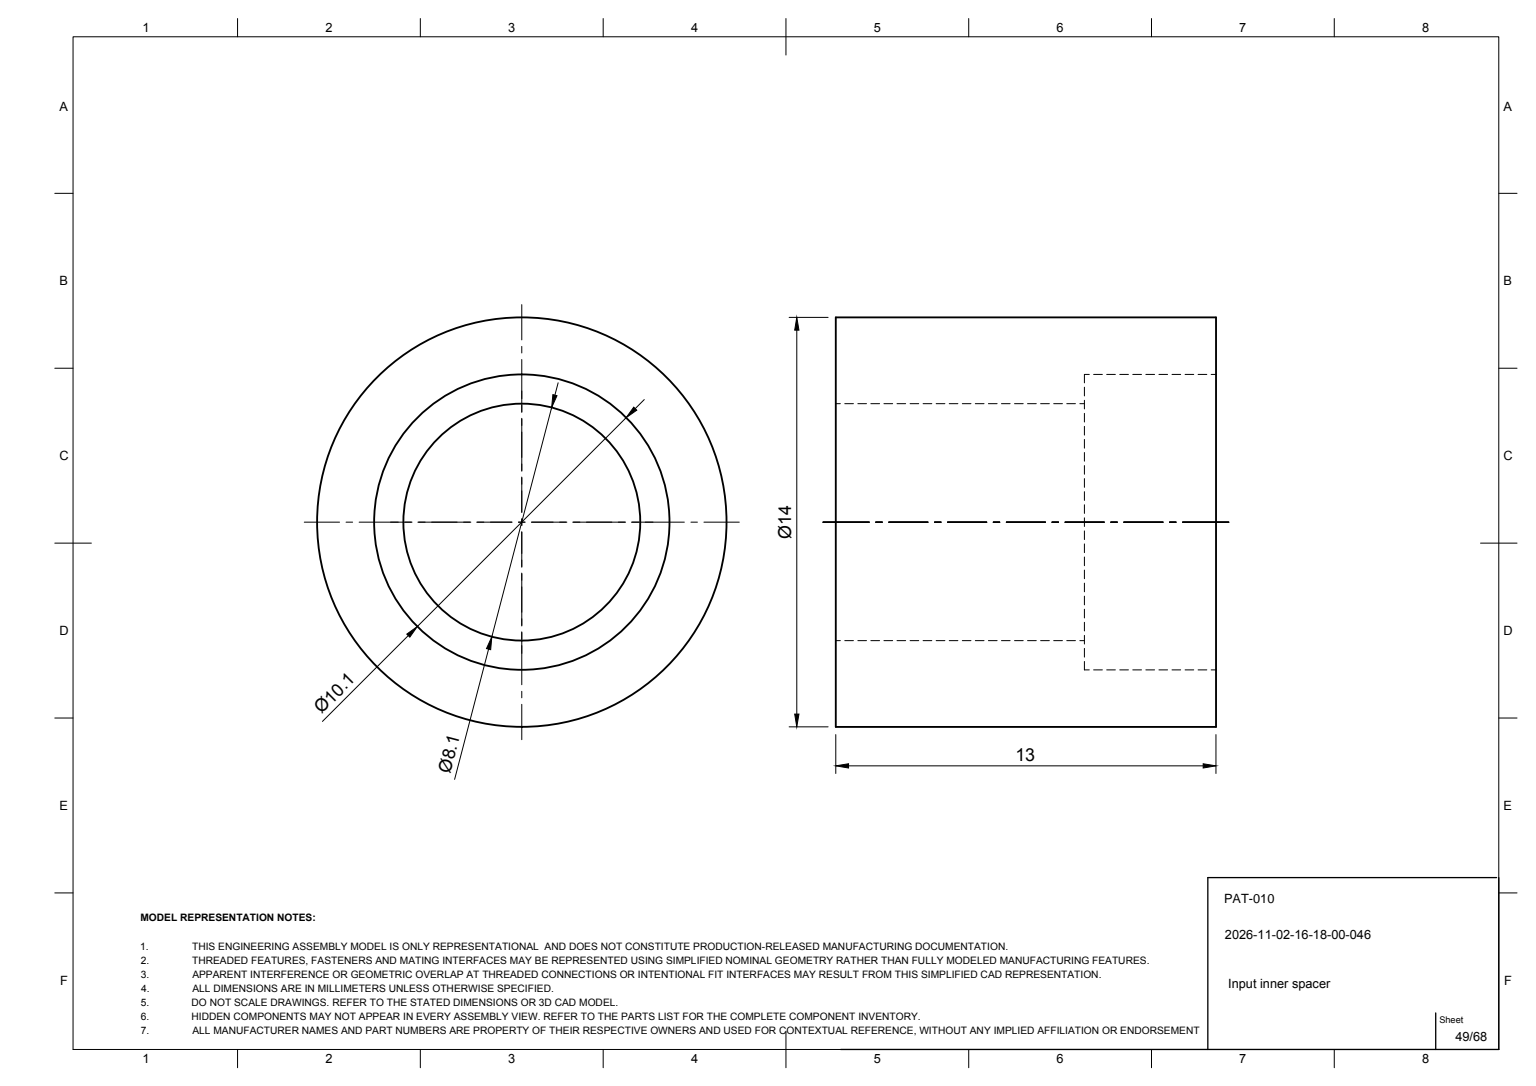
ISO-10303-21;
HEADER;
/* Generated by software containing ST-Developer
 * from STEP Tools, Inc. (www.steptools.com) 
 */

FILE_DESCRIPTION(
/* description */ ('Belt conveyor head drive unit'),
/* implementation_level */ '2;1');

FILE_NAME(
/* name */ 'Input inner spacer.step',
/* time_stamp */ '2026-10-28T03:26:19-07:00',
/* author */ (''),
/* organization */ (''),
/* preprocessor_version */ 'ST-DEVELOPER v20.2',
/* originating_system */ 'Autodesk Translation Framework v15.17.0.0',
/* authorisation */ '');

FILE_SCHEMA (('AUTOMOTIVE_DESIGN { 1 0 10303 214 3 1 1 }'));
ENDSEC;

DATA;
#10=MECHANICAL_DESIGN_GEOMETRIC_PRESENTATION_REPRESENTATION('',(#908),#27069);
#754=SHAPE_REPRESENTATION_RELATIONSHIP('SRR','None',#27402,#823);
#823=ADVANCED_BREP_SHAPE_REPRESENTATION('',(#989),#27044);
#908=STYLED_ITEM('',(#27811),#989);
#989=MANIFOLD_SOLID_BREP('Body1',#13777);
#1209=FACE_BOUND('',#3157,.T.);
#1210=FACE_BOUND('',#3161,.T.);
#1211=FACE_BOUND('',#3163,.T.);
#1547=PLANE('',#15663);
#1548=PLANE('',#15670);
#1549=PLANE('',#15671);
#2158=FACE_OUTER_BOUND('',#3155,.T.);
#2159=FACE_OUTER_BOUND('',#3156,.T.);
#2160=FACE_OUTER_BOUND('',#3158,.T.);
#2161=FACE_OUTER_BOUND('',#3159,.T.);
#2162=FACE_OUTER_BOUND('',#3160,.T.);
#2163=FACE_OUTER_BOUND('',#3162,.T.);
#3155=EDGE_LOOP('',(#11190,#11191,#11192,#11193));
#3156=EDGE_LOOP('',(#11194));
#3157=EDGE_LOOP('',(#11195));
#3158=EDGE_LOOP('',(#11196,#11197,#11198,#11199));
#3159=EDGE_LOOP('',(#11200,#11201,#11202,#11203));
#3160=EDGE_LOOP('',(#11204));
#3161=EDGE_LOOP('',(#11205));
#3162=EDGE_LOOP('',(#11206));
#3163=EDGE_LOOP('',(#11207));
#4049=LINE('',#24483,#4841);
#4050=LINE('',#24490,#4842);
#4051=LINE('',#24496,#4843);
#4841=VECTOR('',#19185,0.505);
#4842=VECTOR('',#19194,0.405);
#4843=VECTOR('',#19201,0.7);
#5591=CIRCLE('',#15661,0.505);
#5592=CIRCLE('',#15662,0.505);
#5593=CIRCLE('',#15664,0.405);
#5594=CIRCLE('',#15666,0.405);
#5595=CIRCLE('',#15668,0.7);
#5596=CIRCLE('',#15669,0.7);
#6717=VERTEX_POINT('',#24480);
#6718=VERTEX_POINT('',#24482);
#6719=VERTEX_POINT('',#24486);
#6720=VERTEX_POINT('',#24489);
#6721=VERTEX_POINT('',#24493);
#6722=VERTEX_POINT('',#24495);
#8287=EDGE_CURVE('',#6717,#6717,#5591,.T.);
#8288=EDGE_CURVE('',#6717,#6718,#4049,.T.);
#8289=EDGE_CURVE('',#6718,#6718,#5592,.T.);
#8290=EDGE_CURVE('',#6719,#6719,#5593,.T.);
#8291=EDGE_CURVE('',#6719,#6720,#4050,.T.);
#8292=EDGE_CURVE('',#6720,#6720,#5594,.T.);
#8293=EDGE_CURVE('',#6721,#6721,#5595,.T.);
#8294=EDGE_CURVE('',#6721,#6722,#4051,.T.);
#8295=EDGE_CURVE('',#6722,#6722,#5596,.T.);
#11190=ORIENTED_EDGE('',*,*,#8287,.F.);
#11191=ORIENTED_EDGE('',*,*,#8288,.T.);
#11192=ORIENTED_EDGE('',*,*,#8289,.F.);
#11193=ORIENTED_EDGE('',*,*,#8288,.F.);
#11194=ORIENTED_EDGE('',*,*,#8287,.T.);
#11195=ORIENTED_EDGE('',*,*,#8290,.F.);
#11196=ORIENTED_EDGE('',*,*,#8290,.T.);
#11197=ORIENTED_EDGE('',*,*,#8291,.T.);
#11198=ORIENTED_EDGE('',*,*,#8292,.T.);
#11199=ORIENTED_EDGE('',*,*,#8291,.F.);
#11200=ORIENTED_EDGE('',*,*,#8293,.F.);
#11201=ORIENTED_EDGE('',*,*,#8294,.T.);
#11202=ORIENTED_EDGE('',*,*,#8295,.T.);
#11203=ORIENTED_EDGE('',*,*,#8294,.F.);
#11204=ORIENTED_EDGE('',*,*,#8293,.T.);
#11205=ORIENTED_EDGE('',*,*,#8289,.T.);
#11206=ORIENTED_EDGE('',*,*,#8295,.F.);
#11207=ORIENTED_EDGE('',*,*,#8292,.F.);
#12729=CYLINDRICAL_SURFACE('',#15660,0.505);
#12730=CYLINDRICAL_SURFACE('',#15665,0.405);
#12731=CYLINDRICAL_SURFACE('',#15667,0.7);
#13437=ADVANCED_FACE('',(#2158),#12729,.F.);
#13438=ADVANCED_FACE('',(#2159,#1209),#1547,.T.);
#13439=ADVANCED_FACE('',(#2160),#12730,.F.);
#13440=ADVANCED_FACE('',(#2161),#12731,.T.);
#13441=ADVANCED_FACE('',(#2162,#1210),#1548,.T.);
#13442=ADVANCED_FACE('',(#2163,#1211),#1549,.F.);
#13777=CLOSED_SHELL('',(#13437,#13438,#13439,#13440,#13441,#13442));
#15659=AXIS2_PLACEMENT_3D('',#24478,#19179,#19180);
#15660=AXIS2_PLACEMENT_3D('',#24479,#19181,#19182);
#15661=AXIS2_PLACEMENT_3D('',#24481,#19183,#19184);
#15662=AXIS2_PLACEMENT_3D('',#24484,#19186,#19187);
#15663=AXIS2_PLACEMENT_3D('',#24485,#19188,#19189);
#15664=AXIS2_PLACEMENT_3D('',#24487,#19190,#19191);
#15665=AXIS2_PLACEMENT_3D('',#24488,#19192,#19193);
#15666=AXIS2_PLACEMENT_3D('',#24491,#19195,#19196);
#15667=AXIS2_PLACEMENT_3D('',#24492,#19197,#19198);
#15668=AXIS2_PLACEMENT_3D('',#24494,#19199,#19200);
#15669=AXIS2_PLACEMENT_3D('',#24497,#19202,#19203);
#15670=AXIS2_PLACEMENT_3D('',#24498,#19204,#19205);
#15671=AXIS2_PLACEMENT_3D('',#24499,#19206,#19207);
#19179=DIRECTION('axis',(0.,0.,1.));
#19180=DIRECTION('refdir',(1.,0.,0.));
#19181=DIRECTION('center_axis',(0.,1.,0.));
#19182=DIRECTION('ref_axis',(1.,0.,0.));
#19183=DIRECTION('center_axis',(0.,1.,0.));
#19184=DIRECTION('ref_axis',(1.,0.,0.));
#19185=DIRECTION('',(0.,1.,0.));
#19186=DIRECTION('center_axis',(0.,-1.,0.));
#19187=DIRECTION('ref_axis',(1.,0.,0.));
#19188=DIRECTION('center_axis',(0.,1.,0.));
#19189=DIRECTION('ref_axis',(1.,0.,0.));
#19190=DIRECTION('center_axis',(0.,1.,0.));
#19191=DIRECTION('ref_axis',(1.,0.,0.));
#19192=DIRECTION('center_axis',(0.,1.,0.));
#19193=DIRECTION('ref_axis',(1.,0.,0.));
#19194=DIRECTION('',(0.,-1.,0.));
#19195=DIRECTION('center_axis',(0.,-1.,0.));
#19196=DIRECTION('ref_axis',(1.,0.,0.));
#19197=DIRECTION('center_axis',(0.,1.,0.));
#19198=DIRECTION('ref_axis',(1.,0.,0.));
#19199=DIRECTION('center_axis',(0.,1.,0.));
#19200=DIRECTION('ref_axis',(1.,0.,0.));
#19201=DIRECTION('',(0.,-1.,0.));
#19202=DIRECTION('center_axis',(0.,1.,0.));
#19203=DIRECTION('ref_axis',(1.,0.,0.));
#19204=DIRECTION('center_axis',(0.,1.,0.));
#19205=DIRECTION('ref_axis',(1.,0.,0.));
#19206=DIRECTION('center_axis',(0.,1.,0.));
#19207=DIRECTION('ref_axis',(1.,0.,0.));
#24478=CARTESIAN_POINT('',(0.,0.,0.));
#24479=CARTESIAN_POINT('Origin',(0.,-1.8,7.));
#24480=CARTESIAN_POINT('',(-0.505,-1.8,7.));
#24481=CARTESIAN_POINT('Origin',(0.,-1.8,7.));
#24482=CARTESIAN_POINT('',(-0.505,-1.35,7.));
#24483=CARTESIAN_POINT('',(-0.505,-1.8,7.));
#24484=CARTESIAN_POINT('Origin',(0.,-1.35,7.));
#24485=CARTESIAN_POINT('Origin',(0.,-1.8,7.));
#24486=CARTESIAN_POINT('',(-0.405,-1.8,7.));
#24487=CARTESIAN_POINT('Origin',(0.,-1.8,7.));
#24488=CARTESIAN_POINT('Origin',(0.,-2.65,7.));
#24489=CARTESIAN_POINT('',(-0.405,-2.65,7.));
#24490=CARTESIAN_POINT('',(-0.405,-2.65,7.));
#24491=CARTESIAN_POINT('Origin',(0.,-2.65,7.));
#24492=CARTESIAN_POINT('Origin',(0.,-2.65,7.));
#24493=CARTESIAN_POINT('',(-0.7,-1.35,7.));
#24494=CARTESIAN_POINT('Origin',(0.,-1.35,7.));
#24495=CARTESIAN_POINT('',(-0.7,-2.65,7.));
#24496=CARTESIAN_POINT('',(-0.7,-2.65,7.));
#24497=CARTESIAN_POINT('Origin',(0.,-2.65,7.));
#24498=CARTESIAN_POINT('Origin',(0.,-1.35,7.));
#24499=CARTESIAN_POINT('Origin',(0.,-2.65,7.));
#26967=UNCERTAINTY_MEASURE_WITH_UNIT(LENGTH_MEASURE(0.001),#27070,
'DISTANCE_ACCURACY_VALUE',
'Maximum model space distance between geometric entities at asserted c
onnectivities');
#26992=UNCERTAINTY_MEASURE_WITH_UNIT(LENGTH_MEASURE(0.001),#27070,
'DISTANCE_ACCURACY_VALUE',
'Maximum model space distance between geometric entities at asserted c
onnectivities');
#27044=(
GEOMETRIC_REPRESENTATION_CONTEXT(3)
GLOBAL_UNCERTAINTY_ASSIGNED_CONTEXT((#26967))
GLOBAL_UNIT_ASSIGNED_CONTEXT((#27070,#27072,#27073))
REPRESENTATION_CONTEXT('','3D')
);
#27069=(
GEOMETRIC_REPRESENTATION_CONTEXT(3)
GLOBAL_UNCERTAINTY_ASSIGNED_CONTEXT((#26992))
GLOBAL_UNIT_ASSIGNED_CONTEXT((#27070,#27072,#27073))
REPRESENTATION_CONTEXT('','3D')
);
#27070=(
LENGTH_UNIT()
NAMED_UNIT(*)
SI_UNIT(.CENTI.,.METRE.)
);
#27072=(
NAMED_UNIT(*)
PLANE_ANGLE_UNIT()
SI_UNIT($,.RADIAN.)
);
#27073=(
NAMED_UNIT(*)
SI_UNIT($,.STERADIAN.)
SOLID_ANGLE_UNIT()
);
#27125=SHAPE_DEFINITION_REPRESENTATION(#27213,#27402);
#27213=PRODUCT_DEFINITION_SHAPE('',$,#27479);
#27402=SHAPE_REPRESENTATION('',(#15659),#27044);
#27427=PRODUCT_DEFINITION_CONTEXT('part definition',#27657,'design');
#27479=PRODUCT_DEFINITION('Input inner spacer','Input inner spacer',#27555,
#27427);
#27555=PRODUCT_DEFINITION_FORMATION('',$,#27710);
#27657=APPLICATION_CONTEXT(
'Core Data for Automotive Mechanical Design Process');
#27658=PRODUCT_CONTEXT('part definition',#27657,'mechanical');
#27710=PRODUCT('Input inner spacer','Input inner spacer',
'Input inner spacer',(#27658));
#27805=COLOUR_RGB('Off White',0.89,0.88,0.83);
#27806=FILL_AREA_STYLE_COLOUR('',#27805);
#27807=FILL_AREA_STYLE('',(#27806));
#27808=SURFACE_STYLE_FILL_AREA(#27807);
#27809=SURFACE_SIDE_STYLE('',(#27808));
#27810=SURFACE_STYLE_USAGE(.BOTH.,#27809);
#27811=PRESENTATION_STYLE_ASSIGNMENT((#27810));
ENDSEC;
END-ISO-10303-21;
